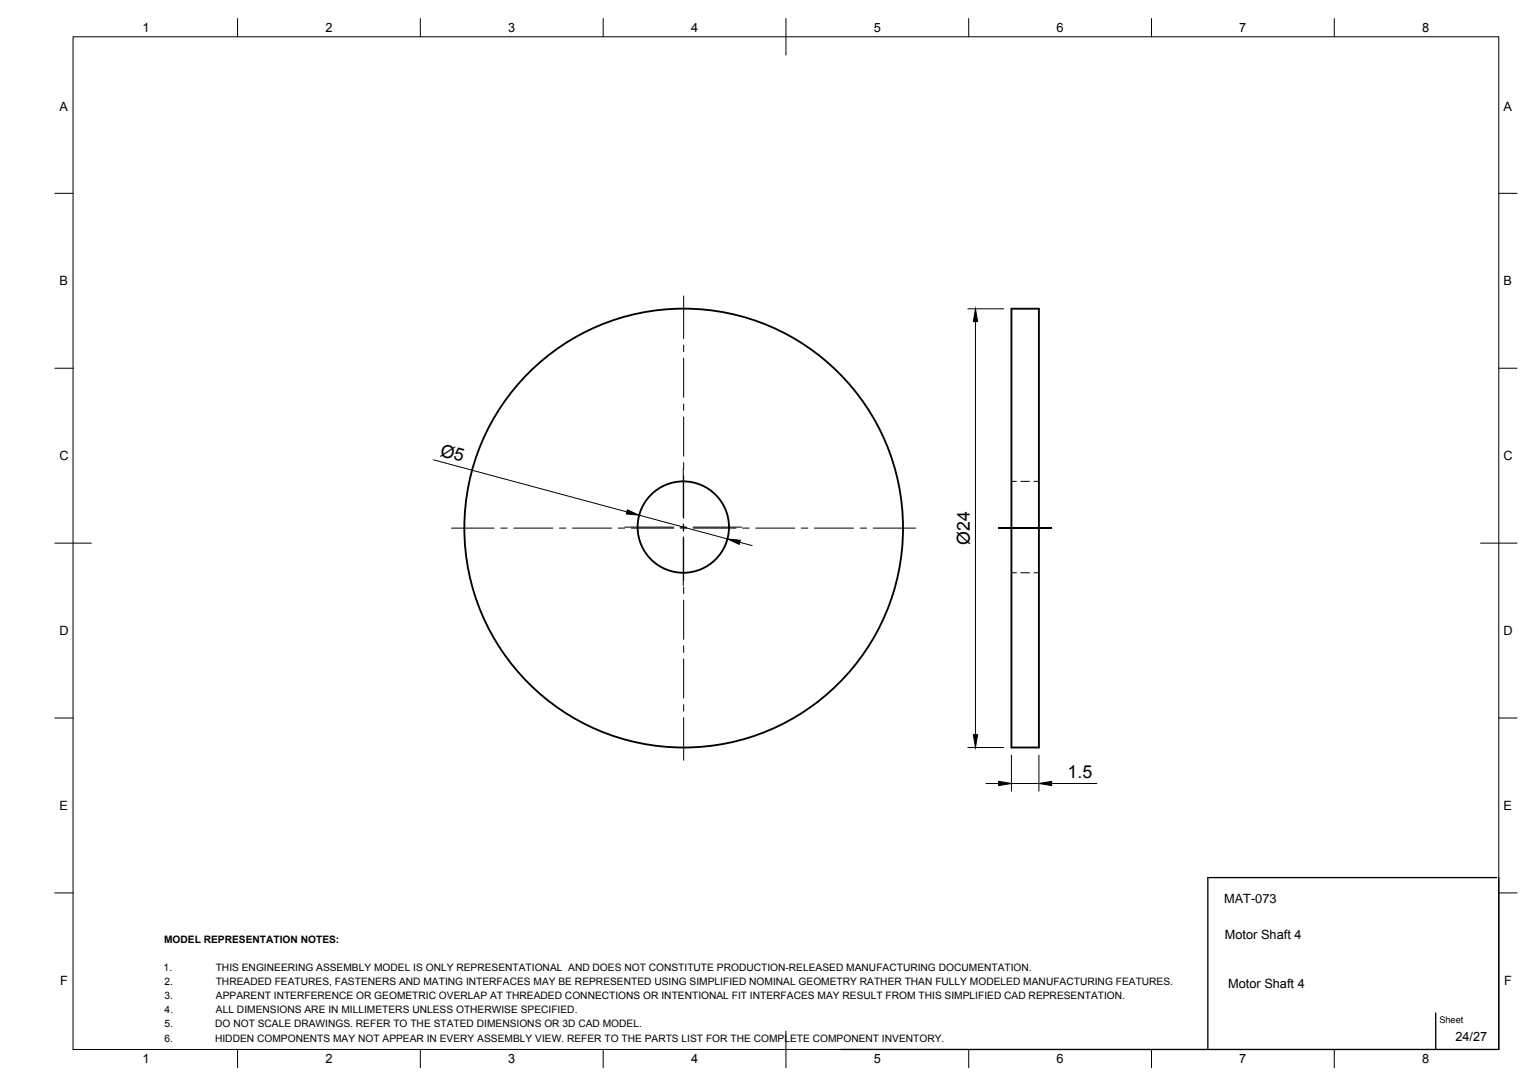
ISO-10303-21;
HEADER;
/* Generated by software containing ST-Developer
 * from STEP Tools, Inc. (www.steptools.com) 
 */

FILE_DESCRIPTION(
/* description */ ('CAx-IF Rec.Pracs.---Representation and Presentation of Product Manufa
cturing Information (PMI)---4.0---2014-10-13'),
/* implementation_level */ '2;1');

FILE_NAME(
/* name */ 'Motor Shaft 4.step',
/* time_stamp */ '2026-10-24T18:52:33-07:00',
/* author */ (''),
/* organization */ (''),
/* preprocessor_version */ 'ST-DEVELOPER v20.2',
/* originating_system */ 'Autodesk Translation Framework v15.17.0.0',
/* authorisation */ '');

FILE_SCHEMA (('AP242_MANAGED_MODEL_BASED_3D_ENGINEERING_MIM_LF { 1 0 10303 442 2 1 4 }'));
ENDSEC;

DATA;
#10=MECHANICAL_DESIGN_GEOMETRIC_PRESENTATION_REPRESENTATION('',(#441),#34876);
#375=SHAPE_REPRESENTATION_RELATIONSHIP('SRR','None',#35012,#408);
#408=ADVANCED_BREP_SHAPE_REPRESENTATION('',(#474),#34870);
#441=STYLED_ITEM('',(#35164),#474);
#474=MANIFOLD_SOLID_BREP('Motor Shaft 4',#19581);
#584=FACE_BOUND('',#6869,.T.);
#585=FACE_BOUND('',#6871,.T.);
#1033=PLANE('',#21966);
#1034=PLANE('',#21967);
#2529=LINE('',#33922,#4128);
#2530=LINE('',#33928,#4129);
#4128=VECTOR('',#27726,0.0025);
#4129=VECTOR('',#27733,0.012);
#4742=CYLINDRICAL_SURFACE('',#21960,0.0025);
#4743=CYLINDRICAL_SURFACE('',#21963,0.012);
#5717=FACE_OUTER_BOUND('',#6866,.T.);
#5718=FACE_OUTER_BOUND('',#6867,.T.);
#5719=FACE_OUTER_BOUND('',#6868,.T.);
#5720=FACE_OUTER_BOUND('',#6870,.T.);
#6866=EDGE_LOOP('',(#17854,#17855,#17856,#17857));
#6867=EDGE_LOOP('',(#17858,#17859,#17860,#17861));
#6868=EDGE_LOOP('',(#17862));
#6869=EDGE_LOOP('',(#17863));
#6870=EDGE_LOOP('',(#17864));
#6871=EDGE_LOOP('',(#17865));
#7937=CIRCLE('',#21961,0.00250000000001);
#7938=CIRCLE('',#21962,0.00250000000001);
#7939=CIRCLE('',#21964,0.01200000000001);
#7940=CIRCLE('',#21965,0.01200000000001);
#9747=VERTEX_POINT('',#33919);
#9748=VERTEX_POINT('',#33921);
#9749=VERTEX_POINT('',#33925);
#9750=VERTEX_POINT('',#33927);
#12485=EDGE_CURVE('',#9747,#9747,#7937,.T.);
#12486=EDGE_CURVE('',#9747,#9748,#2529,.T.);
#12487=EDGE_CURVE('',#9748,#9748,#7938,.T.);
#12488=EDGE_CURVE('',#9749,#9749,#7939,.T.);
#12489=EDGE_CURVE('',#9749,#9750,#2530,.T.);
#12490=EDGE_CURVE('',#9750,#9750,#7940,.T.);
#17854=ORIENTED_EDGE('',*,*,#12485,.T.);
#17855=ORIENTED_EDGE('',*,*,#12486,.T.);
#17856=ORIENTED_EDGE('',*,*,#12487,.T.);
#17857=ORIENTED_EDGE('',*,*,#12486,.F.);
#17858=ORIENTED_EDGE('',*,*,#12488,.T.);
#17859=ORIENTED_EDGE('',*,*,#12489,.T.);
#17860=ORIENTED_EDGE('',*,*,#12490,.T.);
#17861=ORIENTED_EDGE('',*,*,#12489,.F.);
#17862=ORIENTED_EDGE('',*,*,#12490,.F.);
#17863=ORIENTED_EDGE('',*,*,#12485,.F.);
#17864=ORIENTED_EDGE('',*,*,#12488,.F.);
#17865=ORIENTED_EDGE('',*,*,#12487,.F.);
#19433=ADVANCED_FACE('',(#5717),#4742,.F.);
#19434=ADVANCED_FACE('',(#5718),#4743,.T.);
#19435=ADVANCED_FACE('',(#5719,#584),#1033,.F.);
#19436=ADVANCED_FACE('',(#5720,#585),#1034,.T.);
#19581=CLOSED_SHELL('',(#19433,#19434,#19435,#19436));
#21959=AXIS2_PLACEMENT_3D('',#33917,#27720,#27721);
#21960=AXIS2_PLACEMENT_3D('',#33918,#27722,#27723);
#21961=AXIS2_PLACEMENT_3D('',#33920,#27724,#27725);
#21962=AXIS2_PLACEMENT_3D('',#33923,#27727,#27728);
#21963=AXIS2_PLACEMENT_3D('',#33924,#27729,#27730);
#21964=AXIS2_PLACEMENT_3D('',#33926,#27731,#27732);
#21965=AXIS2_PLACEMENT_3D('',#33929,#27734,#27735);
#21966=AXIS2_PLACEMENT_3D('',#33930,#27736,#27737);
#21967=AXIS2_PLACEMENT_3D('',#33931,#27738,#27739);
#27720=DIRECTION('axis',(0.,0.,1.));
#27721=DIRECTION('refdir',(1.,0.,0.));
#27722=DIRECTION('center_axis',(-6.65798752924967E-17,1.,-1.71022579061586E-31));
#27723=DIRECTION('ref_axis',(0.211873077029416,1.41064830464559E-17,-0.97729719084324));
#27724=DIRECTION('center_axis',(6.65798752924967E-17,-1.,1.71022579061586E-31));
#27725=DIRECTION('ref_axis',(0.211873077029416,1.41064830464559E-17,-0.977297190843239));
#27726=DIRECTION('',(-6.65798752924967E-17,1.,-1.71022579061586E-31));
#27727=DIRECTION('center_axis',(-6.65798752924967E-17,1.,-1.71022579061586E-31));
#27728=DIRECTION('ref_axis',(0.211873077029416,1.41064830464559E-17,-0.977297190843239));
#27729=DIRECTION('center_axis',(-6.65798752924967E-17,1.,-1.71022579061586E-31));
#27730=DIRECTION('ref_axis',(-0.211873077029416,-1.41064830464559E-17,0.977297190843239));
#27731=DIRECTION('center_axis',(6.65798752924967E-17,-1.,1.71022579061586E-31));
#27732=DIRECTION('ref_axis',(-0.211873077029416,-1.41064830464559E-17,0.977297190843239));
#27733=DIRECTION('',(6.65798752924967E-17,-1.,1.71022579061586E-31));
#27734=DIRECTION('center_axis',(-6.65798752924967E-17,1.,-1.71022579061586E-31));
#27735=DIRECTION('ref_axis',(-0.211873077029416,-1.41064830464559E-17,0.977297190843239));
#27736=DIRECTION('center_axis',(-6.65798752924967E-17,1.,-1.71022579061586E-31));
#27737=DIRECTION('ref_axis',(-0.211873077029416,-1.41064830464559E-17,0.97729719084324));
#27738=DIRECTION('center_axis',(-6.65798752924967E-17,1.,-1.71022579061586E-31));
#27739=DIRECTION('ref_axis',(-0.211873077029416,-1.41064830464559E-17,0.97729719084324));
#33917=CARTESIAN_POINT('',(0.,0.,0.));
#33918=CARTESIAN_POINT('Origin',(-4.42567805516485E-17,-0.017,1.23897393496637E-32));
#33919=CARTESIAN_POINT('',(-0.000529682692573584,-0.01700000000001,0.0024432429771081));
#33920=CARTESIAN_POINT('Origin',(-4.42567805516478E-17,-0.01700000000001,
1.23897393496654E-32));
#33921=CARTESIAN_POINT('',(-0.000529682692573584,-0.01550000000001,0.0024432429771081));
#33922=CARTESIAN_POINT('',(-0.000529682692573584,-0.017,0.0024432429771081));
#33923=CARTESIAN_POINT('Origin',(-4.43566503645865E-17,-0.01550000000001,
1.21332054810731E-32));
#33924=CARTESIAN_POINT('Origin',(5.68609676360377E-5,-0.017,-2.15928534185712E-5));
#33925=CARTESIAN_POINT('',(0.00259933789198903,-0.01550000000001,-0.0117491591435374));
#33926=CARTESIAN_POINT('Origin',(5.68609676479293E-5,-0.01550000000001,
-2.15928534262255E-5));
#33927=CARTESIAN_POINT('',(0.00259933789198903,-0.01700000000001,-0.0117491591435374));
#33928=CARTESIAN_POINT('',(0.00259933789198903,-0.017,-0.0117491591435374));
#33929=CARTESIAN_POINT('Origin',(5.68609676479294E-5,-0.01700000000001,
-2.15928534262255E-5));
#33930=CARTESIAN_POINT('Origin',(5.68609676360372E-5,-0.017,-2.15928534185708E-5));
#33931=CARTESIAN_POINT('Origin',(5.68609676360371E-5,-0.0155,-2.15928534185708E-5));
#34835=UNCERTAINTY_MEASURE_WITH_UNIT(LENGTH_MEASURE(1.E-5),#34877,
'DISTANCE_ACCURACY_VALUE',
'Maximum model space distance between geometric entities at asserted c
onnectivities');
#34841=UNCERTAINTY_MEASURE_WITH_UNIT(LENGTH_MEASURE(1.E-5),#34877,
'DISTANCE_ACCURACY_VALUE',
'Maximum model space distance between geometric entities at asserted c
onnectivities');
#34870=(
GEOMETRIC_REPRESENTATION_CONTEXT(3)
GLOBAL_UNCERTAINTY_ASSIGNED_CONTEXT((#34835))
GLOBAL_UNIT_ASSIGNED_CONTEXT((#34877,#34878,#34879))
REPRESENTATION_CONTEXT('','3D')
);
#34876=(
GEOMETRIC_REPRESENTATION_CONTEXT(3)
GLOBAL_UNCERTAINTY_ASSIGNED_CONTEXT((#34841))
GLOBAL_UNIT_ASSIGNED_CONTEXT((#34877,#34878,#34879))
REPRESENTATION_CONTEXT('','3D')
);
#34877=(
LENGTH_UNIT()
NAMED_UNIT(*)
SI_UNIT($,.METRE.)
);
#34878=(
NAMED_UNIT(*)
PLANE_ANGLE_UNIT()
SI_UNIT($,.RADIAN.)
);
#34879=(
NAMED_UNIT(*)
SI_UNIT($,.STERADIAN.)
SOLID_ANGLE_UNIT()
);
#34908=SHAPE_DEFINITION_REPRESENTATION(#34942,#35012);
#34942=PRODUCT_DEFINITION_SHAPE('',$,#35047);
#35012=SHAPE_REPRESENTATION('',(#21959),#34870);
#35018=PRODUCT_DEFINITION_CONTEXT('part definition',#35122,'design');
#35047=PRODUCT_DEFINITION('Motor Shaft 4','Motor Shaft 4',#35081,#35018);
#35081=PRODUCT_DEFINITION_FORMATION('',$,#35152);
#35122=APPLICATION_CONTEXT('Managed model based 3d engineering');
#35123=PRODUCT_CONTEXT('part definition',#35122,'mechanical');
#35152=PRODUCT('Motor Shaft 4','Motor Shaft 4',
'LEGAL AND USAGE DISCLAIMER: this Data/Model is provided \X2\201C\X0\A
S IS\X2\201D\X0\ for informational and representational only. It is a 
geometric approximation and is NOT engineered, certified, or guarantee
d for dimensional accuracy, exact tolerances, or production-level prec
ision. Vendor disclaims all implied warranties including fitness for a
 particular purpose. DO NOT USE FOR DIRECT PHYSICAL MANUFACTURING, AUT
OMATED PRODUCTION, OR SAFETY-CRITICAL SYSTEMS without independent engi
neering verification and resolution of any design discrepancies.',(#35123));
#35164=PRESENTATION_STYLE_ASSIGNMENT((#35173));
#35173=SURFACE_STYLE_USAGE(.BOTH.,#35182);
#35182=SURFACE_SIDE_STYLE('',(#35191));
#35191=SURFACE_STYLE_FILL_AREA(#35200);
#35200=FILL_AREA_STYLE('Plastic - Matte (White)',(#35209));
#35209=FILL_AREA_STYLE_COLOUR('Plastic - Matte (White)',#35218);
#35218=COLOUR_RGB('Plastic - Matte (White)',0.964705882352941,0.964705882352941,
0.952941176470588);
ENDSEC;
END-ISO-10303-21;
